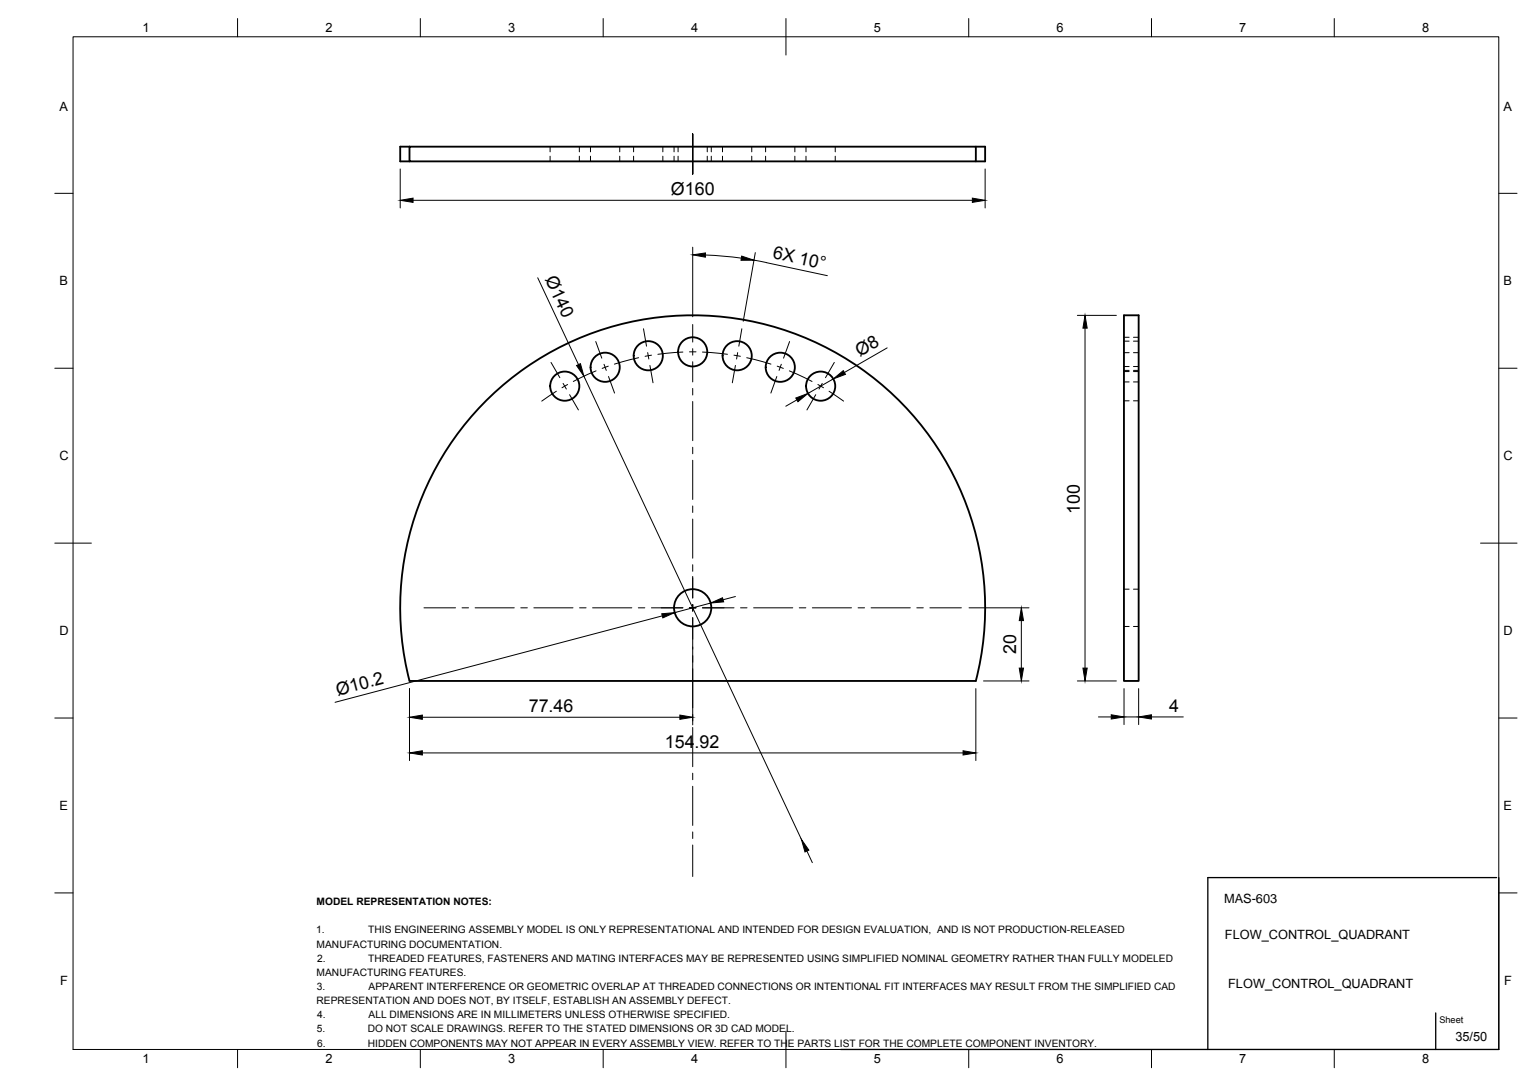
ISO-10303-21;
HEADER;
FILE_DESCRIPTION((''),'2;1');
FILE_NAME('FLOW_CONTROL_QUADRANT.step','2026-10-01T22:06:14-07:00',(''),(''),'','','');
FILE_SCHEMA (('AUTOMOTIVE_DESIGN { 1 0 10303 214 3 1 1 }'));
ENDSEC;
DATA;
#10=MECHANICAL_DESIGN_GEOMETRIC_PRESENTATION_REPRESENTATION('',(#1008),#50440);
#915=SHAPE_REPRESENTATION_RELATIONSHIP('SRR','None',#50648,#960) ;
#960=ADVANCED_BREP_SHAPE_REPRESENTATION('',(#1063),#50417) ;
#1008=STYLED_ITEM('',(#50883),#1063) ;
#1063=MANIFOLD_SOLID_BREP('FLOW_CONTROL_QUADRANT',#28675) ;
#1354=FACE_BOUND('',#5182,.T.) ;
#1355=FACE_BOUND('',#5183,.T.) ;
#1356=FACE_BOUND('',#5184,.T.) ;
#1357=FACE_BOUND('',#5185,.T.) ;
#1358=FACE_BOUND('',#5186,.T.) ;
#1359=FACE_BOUND('',#5187,.T.) ;
#1360=FACE_BOUND('',#5188,.T.) ;
#1361=FACE_BOUND('',#5189,.T.) ;
#1362=FACE_BOUND('',#5191,.T.) ;
#1363=FACE_BOUND('',#5192,.T.) ;
#1364=FACE_BOUND('',#5193,.T.) ;
#1365=FACE_BOUND('',#5194,.T.) ;
#1366=FACE_BOUND('',#5195,.T.) ;
#1367=FACE_BOUND('',#5196,.T.) ;
#1368=FACE_BOUND('',#5197,.T.) ;
#1369=FACE_BOUND('',#5198,.T.) ;
#2205=PLANE('',#30885) ;
#2206=PLANE('',#30886) ;
#2207=PLANE('',#30888) ;
#3376=FACE_OUTER_BOUND('',#5172,.T.) ;
#3377=FACE_OUTER_BOUND('',#5173,.T.) ;
#3378=FACE_OUTER_BOUND('',#5174,.T.) ;
#3379=FACE_OUTER_BOUND('',#5175,.T.) ;
#3380=FACE_OUTER_BOUND('',#5176,.T.) ;
#3381=FACE_OUTER_BOUND('',#5177,.T.) ;
#3382=FACE_OUTER_BOUND('',#5178,.T.) ;
#3383=FACE_OUTER_BOUND('',#5179,.T.) ;
#3384=FACE_OUTER_BOUND('',#5180,.T.) ;
#3385=FACE_OUTER_BOUND('',#5181,.T.) ;
#3386=FACE_OUTER_BOUND('',#5190,.T.) ;
#3387=FACE_OUTER_BOUND('',#5199,.T.) ;
#5172=EDGE_LOOP('',(#23923,#23924,#23925,#23926)) ;
#5173=EDGE_LOOP('',(#23927,#23928,#23929,#23930)) ;
#5174=EDGE_LOOP('',(#23931,#23932,#23933,#23934)) ;
#5175=EDGE_LOOP('',(#23935,#23936,#23937,#23938)) ;
#5176=EDGE_LOOP('',(#23939,#23940,#23941,#23942)) ;
#5177=EDGE_LOOP('',(#23943,#23944,#23945,#23946)) ;
#5178=EDGE_LOOP('',(#23947,#23948,#23949,#23950)) ;
#5179=EDGE_LOOP('',(#23951,#23952,#23953,#23954)) ;
#5180=EDGE_LOOP('',(#23955,#23956,#23957,#23958)) ;
#5181=EDGE_LOOP('',(#23959,#23960)) ;
#5182=EDGE_LOOP('',(#23961)) ;
#5183=EDGE_LOOP('',(#23962)) ;
#5184=EDGE_LOOP('',(#23963)) ;
#5185=EDGE_LOOP('',(#23964)) ;
#5186=EDGE_LOOP('',(#23965)) ;
#5187=EDGE_LOOP('',(#23966)) ;
#5188=EDGE_LOOP('',(#23967)) ;
#5189=EDGE_LOOP('',(#23968)) ;
#5190=EDGE_LOOP('',(#23969,#23970)) ;
#5191=EDGE_LOOP('',(#23971)) ;
#5192=EDGE_LOOP('',(#23972)) ;
#5193=EDGE_LOOP('',(#23973)) ;
#5194=EDGE_LOOP('',(#23974)) ;
#5195=EDGE_LOOP('',(#23975)) ;
#5196=EDGE_LOOP('',(#23976)) ;
#5197=EDGE_LOOP('',(#23977)) ;
#5198=EDGE_LOOP('',(#23978)) ;
#5199=EDGE_LOOP('',(#23979,#23980,#23981,#23982)) ;
#7824=LINE('',#47007,#10296) ;
#7825=LINE('',#47013,#10297) ;
#7826=LINE('',#47019,#10298) ;
#7827=LINE('',#47025,#10299) ;
#7828=LINE('',#47031,#10300) ;
#7829=LINE('',#47037,#10301) ;
#7830=LINE('',#47043,#10302) ;
#7831=LINE('',#47049,#10303) ;
#7832=LINE('',#47054,#10304) ;
#7833=LINE('',#47056,#10305) ;
#7834=LINE('',#47058,#10306) ;
#7835=LINE('',#47059,#10307) ;
#10296=VECTOR('',#37775,0.4) ;
#10297=VECTOR('',#37782,0.4) ;
#10298=VECTOR('',#37789,0.4) ;
#10299=VECTOR('',#37796,0.4) ;
#10300=VECTOR('',#37803,0.4) ;
#10301=VECTOR('',#37810,0.4) ;
#10302=VECTOR('',#37817,0.4) ;
#10303=VECTOR('',#37824,0.51) ;
#10304=VECTOR('',#37829,1.) ;
#10305=VECTOR('',#37830,1.) ;
#10306=VECTOR('',#37831,1.) ;
#10307=VECTOR('',#37832,1.) ;
#11205=CIRCLE('',#30862,0.4) ;
#11206=CIRCLE('',#30863,0.4) ;
#11207=CIRCLE('',#30865,0.4) ;
#11208=CIRCLE('',#30866,0.4) ;
#11209=CIRCLE('',#30868,0.4) ;
#11210=CIRCLE('',#30869,0.4) ;
#11211=CIRCLE('',#30871,0.4) ;
#11212=CIRCLE('',#30872,0.4) ;
#11213=CIRCLE('',#30874,0.4) ;
#11214=CIRCLE('',#30875,0.4) ;
#11215=CIRCLE('',#30877,0.4) ;
#11216=CIRCLE('',#30878,0.4) ;
#11217=CIRCLE('',#30880,0.4) ;
#11218=CIRCLE('',#30881,0.4) ;
#11219=CIRCLE('',#30883,0.51) ;
#11220=CIRCLE('',#30884,0.51) ;
#11221=CIRCLE('',#30887,8.) ;
#11222=CIRCLE('',#30889,8.) ;
#13623=VERTEX_POINT('',#47004) ;
#13624=VERTEX_POINT('',#47006) ;
#13625=VERTEX_POINT('',#47010) ;
#13626=VERTEX_POINT('',#47012) ;
#13627=VERTEX_POINT('',#47016) ;
#13628=VERTEX_POINT('',#47018) ;
#13629=VERTEX_POINT('',#47022) ;
#13630=VERTEX_POINT('',#47024) ;
#13631=VERTEX_POINT('',#47028) ;
#13632=VERTEX_POINT('',#47030) ;
#13633=VERTEX_POINT('',#47034) ;
#13634=VERTEX_POINT('',#47036) ;
#13635=VERTEX_POINT('',#47040) ;
#13636=VERTEX_POINT('',#47042) ;
#13637=VERTEX_POINT('',#47046) ;
#13638=VERTEX_POINT('',#47048) ;
#13639=VERTEX_POINT('',#47052) ;
#13640=VERTEX_POINT('',#47053) ;
#13641=VERTEX_POINT('',#47055) ;
#13642=VERTEX_POINT('',#47057) ;
#17227=EDGE_CURVE('',#13623,#13623,#11205,.T.) ;
#17228=EDGE_CURVE('',#13623,#13624,#7824,.T.) ;
#17229=EDGE_CURVE('',#13624,#13624,#11206,.T.) ;
#17230=EDGE_CURVE('',#13625,#13625,#11207,.T.) ;
#17231=EDGE_CURVE('',#13625,#13626,#7825,.T.) ;
#17232=EDGE_CURVE('',#13626,#13626,#11208,.T.) ;
#17233=EDGE_CURVE('',#13627,#13627,#11209,.T.) ;
#17234=EDGE_CURVE('',#13627,#13628,#7826,.T.) ;
#17235=EDGE_CURVE('',#13628,#13628,#11210,.T.) ;
#17236=EDGE_CURVE('',#13629,#13629,#11211,.T.) ;
#17237=EDGE_CURVE('',#13629,#13630,#7827,.T.) ;
#17238=EDGE_CURVE('',#13630,#13630,#11212,.T.) ;
#17239=EDGE_CURVE('',#13631,#13631,#11213,.T.) ;
#17240=EDGE_CURVE('',#13631,#13632,#7828,.T.) ;
#17241=EDGE_CURVE('',#13632,#13632,#11214,.T.) ;
#17242=EDGE_CURVE('',#13633,#13633,#11215,.T.) ;
#17243=EDGE_CURVE('',#13633,#13634,#7829,.T.) ;
#17244=EDGE_CURVE('',#13634,#13634,#11216,.T.) ;
#17245=EDGE_CURVE('',#13635,#13635,#11217,.T.) ;
#17246=EDGE_CURVE('',#13635,#13636,#7830,.T.) ;
#17247=EDGE_CURVE('',#13636,#13636,#11218,.T.) ;
#17248=EDGE_CURVE('',#13637,#13637,#11219,.T.) ;
#17249=EDGE_CURVE('',#13637,#13638,#7831,.T.) ;
#17250=EDGE_CURVE('',#13638,#13638,#11220,.T.) ;
#17251=EDGE_CURVE('',#13639,#13640,#7832,.T.) ;
#17252=EDGE_CURVE('',#13641,#13639,#7833,.T.) ;
#17253=EDGE_CURVE('',#13642,#13641,#7834,.T.) ;
#17254=EDGE_CURVE('',#13640,#13642,#7835,.T.) ;
#17255=EDGE_CURVE('',#13641,#13642,#11221,.T.) ;
#17256=EDGE_CURVE('',#13640,#13639,#11222,.T.) ;
#23923=ORIENTED_EDGE('',*,*,#17227,.F.) ;
#23924=ORIENTED_EDGE('',*,*,#17228,.T.) ;
#23925=ORIENTED_EDGE('',*,*,#17229,.F.) ;
#23926=ORIENTED_EDGE('',*,*,#17228,.F.) ;
#23927=ORIENTED_EDGE('',*,*,#17230,.F.) ;
#23928=ORIENTED_EDGE('',*,*,#17231,.T.) ;
#23929=ORIENTED_EDGE('',*,*,#17232,.F.) ;
#23930=ORIENTED_EDGE('',*,*,#17231,.F.) ;
#23931=ORIENTED_EDGE('',*,*,#17233,.F.) ;
#23932=ORIENTED_EDGE('',*,*,#17234,.T.) ;
#23933=ORIENTED_EDGE('',*,*,#17235,.F.) ;
#23934=ORIENTED_EDGE('',*,*,#17234,.F.) ;
#23935=ORIENTED_EDGE('',*,*,#17236,.F.) ;
#23936=ORIENTED_EDGE('',*,*,#17237,.T.) ;
#23937=ORIENTED_EDGE('',*,*,#17238,.F.) ;
#23938=ORIENTED_EDGE('',*,*,#17237,.F.) ;
#23939=ORIENTED_EDGE('',*,*,#17239,.F.) ;
#23940=ORIENTED_EDGE('',*,*,#17240,.T.) ;
#23941=ORIENTED_EDGE('',*,*,#17241,.F.) ;
#23942=ORIENTED_EDGE('',*,*,#17240,.F.) ;
#23943=ORIENTED_EDGE('',*,*,#17242,.F.) ;
#23944=ORIENTED_EDGE('',*,*,#17243,.T.) ;
#23945=ORIENTED_EDGE('',*,*,#17244,.F.) ;
#23946=ORIENTED_EDGE('',*,*,#17243,.F.) ;
#23947=ORIENTED_EDGE('',*,*,#17245,.F.) ;
#23948=ORIENTED_EDGE('',*,*,#17246,.T.) ;
#23949=ORIENTED_EDGE('',*,*,#17247,.F.) ;
#23950=ORIENTED_EDGE('',*,*,#17246,.F.) ;
#23951=ORIENTED_EDGE('',*,*,#17248,.F.) ;
#23952=ORIENTED_EDGE('',*,*,#17249,.T.) ;
#23953=ORIENTED_EDGE('',*,*,#17250,.F.) ;
#23954=ORIENTED_EDGE('',*,*,#17249,.F.) ;
#23955=ORIENTED_EDGE('',*,*,#17251,.F.) ;
#23956=ORIENTED_EDGE('',*,*,#17252,.F.) ;
#23957=ORIENTED_EDGE('',*,*,#17253,.F.) ;
#23958=ORIENTED_EDGE('',*,*,#17254,.F.) ;
#23959=ORIENTED_EDGE('',*,*,#17253,.T.) ;
#23960=ORIENTED_EDGE('',*,*,#17255,.T.) ;
#23961=ORIENTED_EDGE('',*,*,#17250,.T.) ;
#23962=ORIENTED_EDGE('',*,*,#17247,.T.) ;
#23963=ORIENTED_EDGE('',*,*,#17244,.T.) ;
#23964=ORIENTED_EDGE('',*,*,#17241,.T.) ;
#23965=ORIENTED_EDGE('',*,*,#17238,.T.) ;
#23966=ORIENTED_EDGE('',*,*,#17235,.T.) ;
#23967=ORIENTED_EDGE('',*,*,#17232,.T.) ;
#23968=ORIENTED_EDGE('',*,*,#17229,.T.) ;
#23969=ORIENTED_EDGE('',*,*,#17251,.T.) ;
#23970=ORIENTED_EDGE('',*,*,#17256,.T.) ;
#23971=ORIENTED_EDGE('',*,*,#17248,.T.) ;
#23972=ORIENTED_EDGE('',*,*,#17245,.T.) ;
#23973=ORIENTED_EDGE('',*,*,#17242,.T.) ;
#23974=ORIENTED_EDGE('',*,*,#17239,.T.) ;
#23975=ORIENTED_EDGE('',*,*,#17236,.T.) ;
#23976=ORIENTED_EDGE('',*,*,#17233,.T.) ;
#23977=ORIENTED_EDGE('',*,*,#17230,.T.) ;
#23978=ORIENTED_EDGE('',*,*,#17227,.T.) ;
#23979=ORIENTED_EDGE('',*,*,#17254,.T.) ;
#23980=ORIENTED_EDGE('',*,*,#17255,.F.) ;
#23981=ORIENTED_EDGE('',*,*,#17252,.T.) ;
#23982=ORIENTED_EDGE('',*,*,#17256,.F.) ;
#26856=CYLINDRICAL_SURFACE('',#30861,0.4) ;
#26857=CYLINDRICAL_SURFACE('',#30864,0.4) ;
#26858=CYLINDRICAL_SURFACE('',#30867,0.4) ;
#26859=CYLINDRICAL_SURFACE('',#30870,0.4) ;
#26860=CYLINDRICAL_SURFACE('',#30873,0.4) ;
#26861=CYLINDRICAL_SURFACE('',#30876,0.4) ;
#26862=CYLINDRICAL_SURFACE('',#30879,0.4) ;
#26863=CYLINDRICAL_SURFACE('',#30882,0.51) ;
#26864=CYLINDRICAL_SURFACE('',#30890,8.) ;
#28111=ADVANCED_FACE('',(#3376),#26856,.F.) ;
#28112=ADVANCED_FACE('',(#3377),#26857,.F.) ;
#28113=ADVANCED_FACE('',(#3378),#26858,.F.) ;
#28114=ADVANCED_FACE('',(#3379),#26859,.F.) ;
#28115=ADVANCED_FACE('',(#3380),#26860,.F.) ;
#28116=ADVANCED_FACE('',(#3381),#26861,.F.) ;
#28117=ADVANCED_FACE('',(#3382),#26862,.F.) ;
#28118=ADVANCED_FACE('',(#3383),#26863,.F.) ;
#28119=ADVANCED_FACE('',(#3384),#2205,.F.) ;
#28120=ADVANCED_FACE('',(#3385,#1354,#1355,#1356,#1357,#1358,#1359,#1360,
#1361),#2206,.T.) ;
#28121=ADVANCED_FACE('',(#3386,#1362,#1363,#1364,#1365,#1366,#1367,#1368,
#1369),#2207,.T.) ;
#28122=ADVANCED_FACE('',(#3387),#26864,.T.) ;
#28675=CLOSED_SHELL('',(#28111,#28112,#28113,#28114,#28115,#28116,#28117,
#28118,#28119,#28120,#28121,#28122)) ;
#30860=AXIS2_PLACEMENT_3D('',#47002,#37769,#37770) ;
#30861=AXIS2_PLACEMENT_3D('',#47003,#37771,#37772) ;
#30862=AXIS2_PLACEMENT_3D('',#47005,#37773,#37774) ;
#30863=AXIS2_PLACEMENT_3D('',#47008,#37776,#37777) ;
#30864=AXIS2_PLACEMENT_3D('',#47009,#37778,#37779) ;
#30865=AXIS2_PLACEMENT_3D('',#47011,#37780,#37781) ;
#30866=AXIS2_PLACEMENT_3D('',#47014,#37783,#37784) ;
#30867=AXIS2_PLACEMENT_3D('',#47015,#37785,#37786) ;
#30868=AXIS2_PLACEMENT_3D('',#47017,#37787,#37788) ;
#30869=AXIS2_PLACEMENT_3D('',#47020,#37790,#37791) ;
#30870=AXIS2_PLACEMENT_3D('',#47021,#37792,#37793) ;
#30871=AXIS2_PLACEMENT_3D('',#47023,#37794,#37795) ;
#30872=AXIS2_PLACEMENT_3D('',#47026,#37797,#37798) ;
#30873=AXIS2_PLACEMENT_3D('',#47027,#37799,#37800) ;
#30874=AXIS2_PLACEMENT_3D('',#47029,#37801,#37802) ;
#30875=AXIS2_PLACEMENT_3D('',#47032,#37804,#37805) ;
#30876=AXIS2_PLACEMENT_3D('',#47033,#37806,#37807) ;
#30877=AXIS2_PLACEMENT_3D('',#47035,#37808,#37809) ;
#30878=AXIS2_PLACEMENT_3D('',#47038,#37811,#37812) ;
#30879=AXIS2_PLACEMENT_3D('',#47039,#37813,#37814) ;
#30880=AXIS2_PLACEMENT_3D('',#47041,#37815,#37816) ;
#30881=AXIS2_PLACEMENT_3D('',#47044,#37818,#37819) ;
#30882=AXIS2_PLACEMENT_3D('',#47045,#37820,#37821) ;
#30883=AXIS2_PLACEMENT_3D('',#47047,#37822,#37823) ;
#30884=AXIS2_PLACEMENT_3D('',#47050,#37825,#37826) ;
#30885=AXIS2_PLACEMENT_3D('',#47051,#37827,#37828) ;
#30886=AXIS2_PLACEMENT_3D('',#47060,#37833,#37834) ;
#30887=AXIS2_PLACEMENT_3D('',#47061,#37835,#37836) ;
#30888=AXIS2_PLACEMENT_3D('',#47062,#37837,#37838) ;
#30889=AXIS2_PLACEMENT_3D('',#47063,#37839,#37840) ;
#30890=AXIS2_PLACEMENT_3D('',#47064,#37841,#37842) ;
#37769=DIRECTION('axis',(0.,0.,1.)) ;
#37770=DIRECTION('refdir',(1.,0.,0.)) ;
#37771=DIRECTION('center_axis',(0.,1.,0.)) ;
#37772=DIRECTION('ref_axis',(1.,0.,0.)) ;
#37773=DIRECTION('center_axis',(0.,1.,0.)) ;
#37774=DIRECTION('ref_axis',(1.,0.,0.)) ;
#37775=DIRECTION('',(0.,1.,0.)) ;
#37776=DIRECTION('center_axis',(0.,-1.,0.)) ;
#37777=DIRECTION('ref_axis',(1.,0.,0.)) ;
#37778=DIRECTION('center_axis',(0.,1.,0.)) ;
#37779=DIRECTION('ref_axis',(1.,0.,0.)) ;
#37780=DIRECTION('center_axis',(0.,1.,0.)) ;
#37781=DIRECTION('ref_axis',(1.,0.,0.)) ;
#37782=DIRECTION('',(0.,1.,0.)) ;
#37783=DIRECTION('center_axis',(0.,-1.,0.)) ;
#37784=DIRECTION('ref_axis',(1.,0.,0.)) ;
#37785=DIRECTION('center_axis',(0.,1.,0.)) ;
#37786=DIRECTION('ref_axis',(1.,0.,0.)) ;
#37787=DIRECTION('center_axis',(0.,1.,0.)) ;
#37788=DIRECTION('ref_axis',(1.,0.,0.)) ;
#37789=DIRECTION('',(0.,1.,0.)) ;
#37790=DIRECTION('center_axis',(0.,-1.,0.)) ;
#37791=DIRECTION('ref_axis',(1.,0.,0.)) ;
#37792=DIRECTION('center_axis',(0.,1.,0.)) ;
#37793=DIRECTION('ref_axis',(1.,0.,0.)) ;
#37794=DIRECTION('center_axis',(0.,1.,0.)) ;
#37795=DIRECTION('ref_axis',(1.,0.,0.)) ;
#37796=DIRECTION('',(0.,1.,0.)) ;
#37797=DIRECTION('center_axis',(0.,-1.,0.)) ;
#37798=DIRECTION('ref_axis',(1.,0.,0.)) ;
#37799=DIRECTION('center_axis',(0.,1.,0.)) ;
#37800=DIRECTION('ref_axis',(1.,0.,0.)) ;
#37801=DIRECTION('center_axis',(0.,1.,0.)) ;
#37802=DIRECTION('ref_axis',(1.,0.,0.)) ;
#37803=DIRECTION('',(0.,1.,0.)) ;
#37804=DIRECTION('center_axis',(0.,-1.,0.)) ;
#37805=DIRECTION('ref_axis',(1.,0.,0.)) ;
#37806=DIRECTION('center_axis',(0.,1.,0.)) ;
#37807=DIRECTION('ref_axis',(1.,0.,0.)) ;
#37808=DIRECTION('center_axis',(0.,1.,0.)) ;
#37809=DIRECTION('ref_axis',(1.,0.,0.)) ;
#37810=DIRECTION('',(0.,1.,0.)) ;
#37811=DIRECTION('center_axis',(0.,-1.,0.)) ;
#37812=DIRECTION('ref_axis',(1.,0.,0.)) ;
#37813=DIRECTION('center_axis',(0.,1.,0.)) ;
#37814=DIRECTION('ref_axis',(1.,0.,0.)) ;
#37815=DIRECTION('center_axis',(0.,1.,0.)) ;
#37816=DIRECTION('ref_axis',(1.,0.,0.)) ;
#37817=DIRECTION('',(0.,1.,0.)) ;
#37818=DIRECTION('center_axis',(0.,-1.,0.)) ;
#37819=DIRECTION('ref_axis',(1.,0.,0.)) ;
#37820=DIRECTION('center_axis',(0.,1.,0.)) ;
#37821=DIRECTION('ref_axis',(1.,0.,0.)) ;
#37822=DIRECTION('center_axis',(0.,1.,0.)) ;
#37823=DIRECTION('ref_axis',(1.,0.,0.)) ;
#37824=DIRECTION('',(0.,1.,0.)) ;
#37825=DIRECTION('center_axis',(0.,-1.,0.)) ;
#37826=DIRECTION('ref_axis',(1.,0.,0.)) ;
#37827=DIRECTION('center_axis',(0.,0.,1.)) ;
#37828=DIRECTION('ref_axis',(1.,0.,0.)) ;
#37829=DIRECTION('',(1.,0.,0.)) ;
#37830=DIRECTION('',(0.,-1.,0.)) ;
#37831=DIRECTION('',(-1.,0.,0.)) ;
#37832=DIRECTION('',(0.,1.,0.)) ;
#37833=DIRECTION('center_axis',(0.,1.,0.)) ;
#37834=DIRECTION('ref_axis',(1.,0.,0.)) ;
#37835=DIRECTION('center_axis',(0.,1.,0.)) ;
#37836=DIRECTION('ref_axis',(1.,0.,0.)) ;
#37837=DIRECTION('center_axis',(0.,-1.,0.)) ;
#37838=DIRECTION('ref_axis',(-1.,0.,0.)) ;
#37839=DIRECTION('center_axis',(0.,-1.,0.)) ;
#37840=DIRECTION('ref_axis',(1.,0.,0.)) ;
#37841=DIRECTION('center_axis',(0.,1.,0.)) ;
#37842=DIRECTION('ref_axis',(6.12323399573677E-17,0.,1.)) ;
#47002=CARTESIAN_POINT('',(0.,0.,0.)) ;
#47003=CARTESIAN_POINT('Origin',(-56.5,18.2,98.0621778264911)) ;
#47004=CARTESIAN_POINT('',(-56.9,18.,98.0621778264911)) ;
#47005=CARTESIAN_POINT('Origin',(-56.5,18.,98.0621778264911)) ;
#47006=CARTESIAN_POINT('',(-56.9,18.4,98.0621778264911)) ;
#47007=CARTESIAN_POINT('',(-56.9,18.2,98.0621778264911)) ;
#47008=CARTESIAN_POINT('Origin',(-56.5,18.4,98.0621778264911)) ;
#47009=CARTESIAN_POINT('Origin',(-55.3941410032797,18.2,98.5778483455014)) ;
#47010=CARTESIAN_POINT('',(-55.7941410032797,18.,98.5778483455014)) ;
#47011=CARTESIAN_POINT('Origin',(-55.3941410032797,18.,98.5778483455014)) ;
#47012=CARTESIAN_POINT('',(-55.7941410032797,18.4,98.5778483455014)) ;
#47013=CARTESIAN_POINT('',(-55.7941410032797,18.2,98.5778483455014)) ;
#47014=CARTESIAN_POINT('Origin',(-55.3941410032797,18.4,98.5778483455014)) ;
#47015=CARTESIAN_POINT('Origin',(-54.2155372436685,18.2,98.8936542710855)) ;
#47016=CARTESIAN_POINT('',(-54.6155372436685,18.,98.8936542710855)) ;
#47017=CARTESIAN_POINT('Origin',(-54.2155372436685,18.,98.8936542710855)) ;
#47018=CARTESIAN_POINT('',(-54.6155372436685,18.4,98.8936542710855)) ;
#47019=CARTESIAN_POINT('',(-54.6155372436685,18.2,98.8936542710855)) ;
#47020=CARTESIAN_POINT('Origin',(-54.2155372436685,18.4,98.8936542710855)) ;
#47021=CARTESIAN_POINT('Origin',(-53.,18.2,99.)) ;
#47022=CARTESIAN_POINT('',(-53.4,18.,99.)) ;
#47023=CARTESIAN_POINT('Origin',(-53.,18.,99.)) ;
#47024=CARTESIAN_POINT('',(-53.4,18.4,99.)) ;
#47025=CARTESIAN_POINT('',(-53.4,18.2,99.)) ;
#47026=CARTESIAN_POINT('Origin',(-53.,18.4,99.)) ;
#47027=CARTESIAN_POINT('Origin',(-51.7844627563315,18.2,98.8936542710855)) ;
#47028=CARTESIAN_POINT('',(-52.1844627563315,18.,98.8936542710855)) ;
#47029=CARTESIAN_POINT('Origin',(-51.7844627563315,18.,98.8936542710855)) ;
#47030=CARTESIAN_POINT('',(-52.1844627563315,18.4,98.8936542710855)) ;
#47031=CARTESIAN_POINT('',(-52.1844627563315,18.2,98.8936542710855)) ;
#47032=CARTESIAN_POINT('Origin',(-51.7844627563315,18.4,98.8936542710855)) ;
#47033=CARTESIAN_POINT('Origin',(-50.6058589967203,18.2,98.5778483455014)) ;
#47034=CARTESIAN_POINT('',(-51.0058589967203,18.,98.5778483455014)) ;
#47035=CARTESIAN_POINT('Origin',(-50.6058589967203,18.,98.5778483455014)) ;
#47036=CARTESIAN_POINT('',(-51.0058589967203,18.4,98.5778483455014)) ;
#47037=CARTESIAN_POINT('',(-51.0058589967203,18.2,98.5778483455014)) ;
#47038=CARTESIAN_POINT('Origin',(-50.6058589967203,18.4,98.5778483455014)) ;
#47039=CARTESIAN_POINT('Origin',(-49.5,18.2,98.0621778264911)) ;
#47040=CARTESIAN_POINT('',(-49.9,18.,98.0621778264911)) ;
#47041=CARTESIAN_POINT('Origin',(-49.5,18.,98.0621778264911)) ;
#47042=CARTESIAN_POINT('',(-49.9,18.4,98.0621778264911)) ;
#47043=CARTESIAN_POINT('',(-49.9,18.2,98.0621778264911)) ;
#47044=CARTESIAN_POINT('Origin',(-49.5,18.4,98.0621778264911)) ;
#47045=CARTESIAN_POINT('Origin',(-53.,18.2,92.)) ;
#47046=CARTESIAN_POINT('',(-53.51,18.,92.)) ;
#47047=CARTESIAN_POINT('Origin',(-53.,18.,92.)) ;
#47048=CARTESIAN_POINT('',(-53.51,18.4,92.)) ;
#47049=CARTESIAN_POINT('',(-53.51,18.2,92.)) ;
#47050=CARTESIAN_POINT('Origin',(-53.,18.4,92.)) ;
#47051=CARTESIAN_POINT('Origin',(-53.,18.2,90.)) ;
#47052=CARTESIAN_POINT('',(-60.7459666924148,18.,90.)) ;
#47053=CARTESIAN_POINT('',(-45.2540333075852,18.,90.)) ;
#47054=CARTESIAN_POINT('',(-53.,18.,90.)) ;
#47055=CARTESIAN_POINT('',(-60.7459666924148,18.4,90.)) ;
#47056=CARTESIAN_POINT('',(-60.7459666924148,18.2,90.)) ;
#47057=CARTESIAN_POINT('',(-45.2540333075852,18.4,90.)) ;
#47058=CARTESIAN_POINT('',(-53.,18.4,90.)) ;
#47059=CARTESIAN_POINT('',(-45.2540333075852,18.2,90.)) ;
#47060=CARTESIAN_POINT('Origin',(-53.,18.4,92.)) ;
#47061=CARTESIAN_POINT('Origin',(-53.,18.4,92.)) ;
#47062=CARTESIAN_POINT('Origin',(-53.,18.,92.)) ;
#47063=CARTESIAN_POINT('Origin',(-53.,18.,92.)) ;
#47064=CARTESIAN_POINT('Origin',(-53.,18.2,92.)) ;
#50364=UNCERTAINTY_MEASURE_WITH_UNIT(LENGTH_MEASURE(0.001),#50441,
'DISTANCE_ACCURACY_VALUE',
'Maximum model space distance between geometric entities at asserted c
onnectivities') ;
#50387=UNCERTAINTY_MEASURE_WITH_UNIT(LENGTH_MEASURE(0.001),#50441,
'DISTANCE_ACCURACY_VALUE',
'Maximum model space distance between geometric entities at asserted c
onnectivities') ;
#50417=(
GEOMETRIC_REPRESENTATION_CONTEXT(3)
GLOBAL_UNCERTAINTY_ASSIGNED_CONTEXT((#50364))
GLOBAL_UNIT_ASSIGNED_CONTEXT((#50441,#50443,#50444))
REPRESENTATION_CONTEXT('','3D')
) ;
#50440=(
GEOMETRIC_REPRESENTATION_CONTEXT(3)
GLOBAL_UNCERTAINTY_ASSIGNED_CONTEXT((#50387))
GLOBAL_UNIT_ASSIGNED_CONTEXT((#50441,#50443,#50444))
REPRESENTATION_CONTEXT('','3D')
) ;
#50441=(
LENGTH_UNIT()
NAMED_UNIT(*)
SI_UNIT(.CENTI.,.METRE.)
) ;
#50443=(
NAMED_UNIT(*)
PLANE_ANGLE_UNIT()
SI_UNIT($,.RADIAN.)
) ;
#50444=(
NAMED_UNIT(*)
SI_UNIT($,.STERADIAN.)
SOLID_ANGLE_UNIT()
) ;
#50474=SHAPE_DEFINITION_REPRESENTATION(#50550,#50648) ;
#50550=PRODUCT_DEFINITION_SHAPE('',$,#50701) ;
#50648=SHAPE_REPRESENTATION('',(#30860),#50417) ;
#50671=PRODUCT_DEFINITION_CONTEXT('part definition',#50829,'design') ;
#50701=PRODUCT_DEFINITION('FLOW_CONTROL_QUADRANT',
'FLOW_CONTROL_QUADRANT',#50753,#50671) ;
#50753=PRODUCT_DEFINITION_FORMATION('',$,#50860) ;
#50829=APPLICATION_CONTEXT(
'Core Data for Automotive Mechanical Design Process') ;
#50830=PRODUCT_CONTEXT('part definition',#50829,'mechanical') ;
#50860=PRODUCT('FLOW_CONTROL_QUADRANT','FLOW_CONTROL_QUADRANT',$,(#50830)) ;
#50883=PRESENTATION_STYLE_ASSIGNMENT((#50890)) ;
#50890=SURFACE_STYLE_USAGE(.BOTH.,#50897) ;
#50897=SURFACE_SIDE_STYLE('',(#50904)) ;
#50904=SURFACE_STYLE_FILL_AREA(#50911) ;
#50911=FILL_AREA_STYLE('Steel - Satin',(#50918)) ;
#50918=FILL_AREA_STYLE_COLOUR('Steel - Satin',#50925) ;
#50925=COLOUR_RGB('Steel - Satin', 0.31764706, 0.68627451, 0.89019608) ;
ENDSEC;
END-ISO-10303-21;
